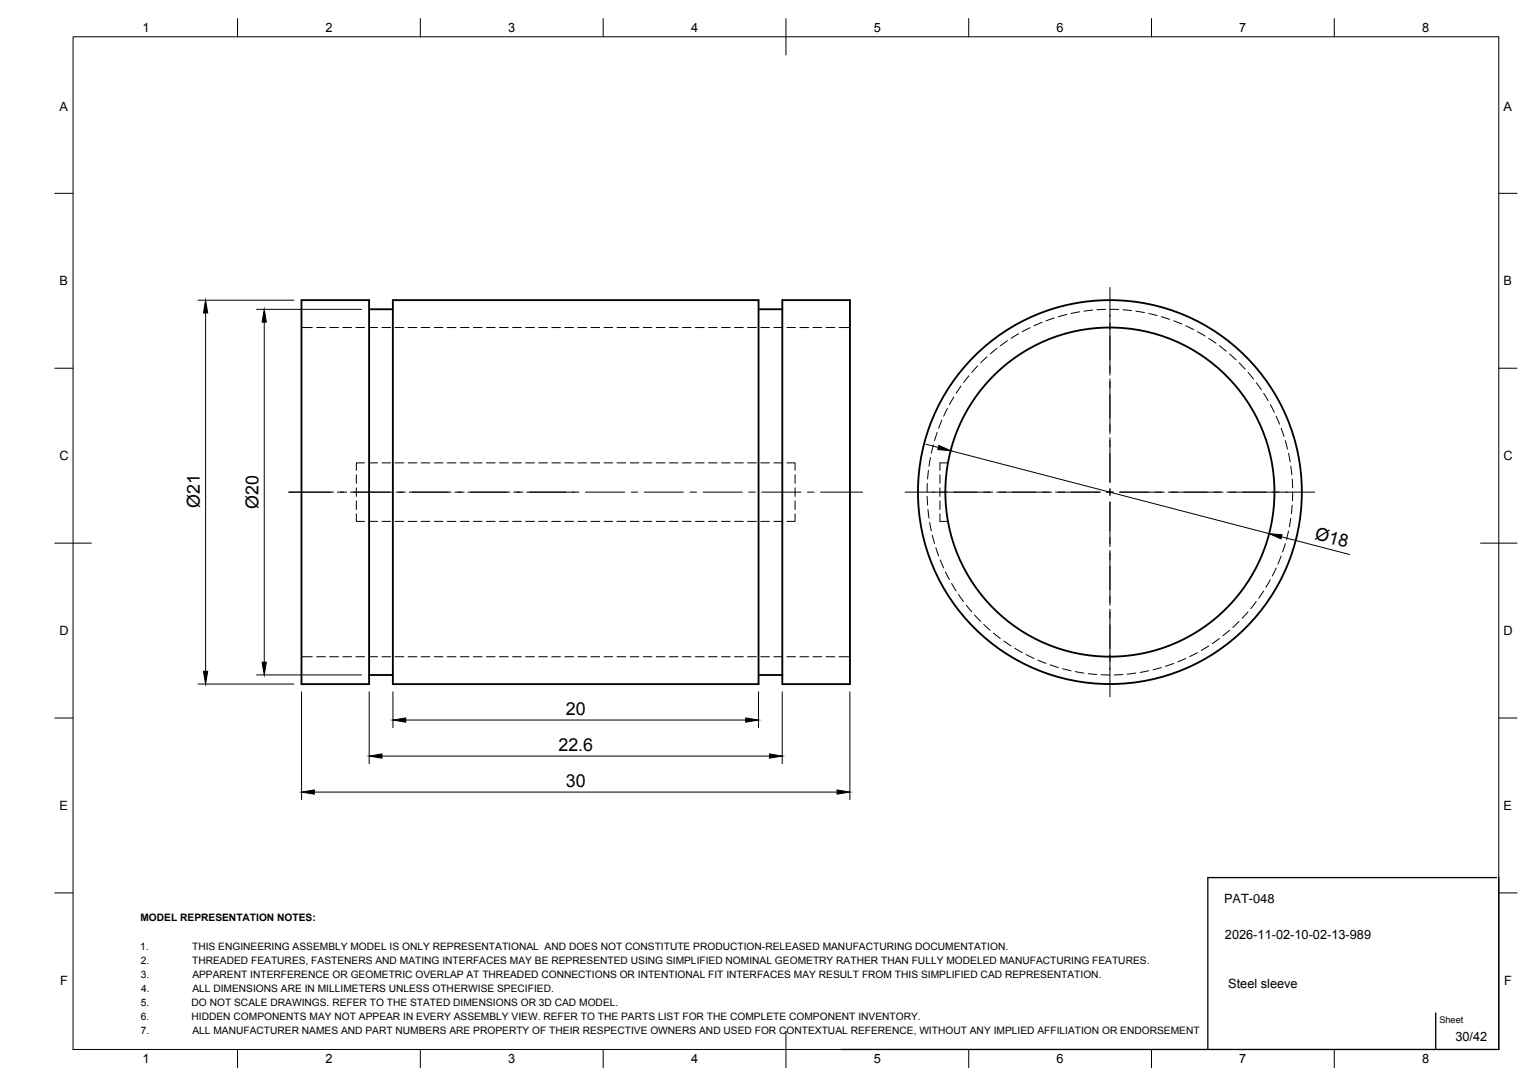
ISO-10303-21;
HEADER;
/* Generated by software containing ST-Developer
 * from STEP Tools, Inc. (www.steptools.com) 
 */

FILE_DESCRIPTION(
/* description */ ('Guided pneumatic stop gate'),
/* implementation_level */ '2;1');

FILE_NAME(
/* name */ 'Steel sleeve.step',
/* time_stamp */ '2026-10-27T21:43:45-07:00',
/* author */ (''),
/* organization */ (''),
/* preprocessor_version */ 'ST-DEVELOPER v20.2',
/* originating_system */ 'Autodesk Translation Framework v15.17.0.0',
/* authorisation */ '');

FILE_SCHEMA (('AUTOMOTIVE_DESIGN { 1 0 10303 214 3 1 1 }'));
ENDSEC;

DATA;
#10=MECHANICAL_DESIGN_GEOMETRIC_PRESENTATION_REPRESENTATION('',(#559),#14392);
#475=SHAPE_REPRESENTATION_RELATIONSHIP('SRR','None',#14611,#517);
#517=ADVANCED_BREP_SHAPE_REPRESENTATION('',(#600),#14373);
#559=STYLED_ITEM('',(#14905),#600);
#600=MANIFOLD_SOLID_BREP('Body1',#7900);
#777=FACE_BOUND('',#2059,.T.);
#778=FACE_BOUND('',#2062,.T.);
#779=FACE_BOUND('',#2065,.T.);
#780=FACE_BOUND('',#2068,.T.);
#781=FACE_BOUND('',#2071,.T.);
#782=FACE_BOUND('',#2074,.T.);
#783=FACE_BOUND('',#2076,.T.);
#1003=PLANE('',#8982);
#1004=PLANE('',#8984);
#1005=PLANE('',#8985);
#1006=PLANE('',#8987);
#1007=PLANE('',#8988);
#1008=PLANE('',#8989);
#1009=PLANE('',#8994);
#1010=PLANE('',#8998);
#1011=PLANE('',#9002);
#1012=PLANE('',#9006);
#1013=PLANE('',#9010);
#1416=FACE_OUTER_BOUND('',#2053,.T.);
#1417=FACE_OUTER_BOUND('',#2054,.T.);
#1418=FACE_OUTER_BOUND('',#2055,.T.);
#1419=FACE_OUTER_BOUND('',#2056,.T.);
#1420=FACE_OUTER_BOUND('',#2057,.T.);
#1421=FACE_OUTER_BOUND('',#2058,.T.);
#1422=FACE_OUTER_BOUND('',#2060,.T.);
#1423=FACE_OUTER_BOUND('',#2061,.T.);
#1424=FACE_OUTER_BOUND('',#2063,.T.);
#1425=FACE_OUTER_BOUND('',#2064,.T.);
#1426=FACE_OUTER_BOUND('',#2066,.T.);
#1427=FACE_OUTER_BOUND('',#2067,.T.);
#1428=FACE_OUTER_BOUND('',#2069,.T.);
#1429=FACE_OUTER_BOUND('',#2070,.T.);
#1430=FACE_OUTER_BOUND('',#2072,.T.);
#1431=FACE_OUTER_BOUND('',#2073,.T.);
#1432=FACE_OUTER_BOUND('',#2075,.T.);
#2053=EDGE_LOOP('',(#6546,#6547,#6548,#6549));
#2054=EDGE_LOOP('',(#6550,#6551,#6552,#6553));
#2055=EDGE_LOOP('',(#6554,#6555,#6556,#6557));
#2056=EDGE_LOOP('',(#6558,#6559,#6560,#6561));
#2057=EDGE_LOOP('',(#6562,#6563,#6564,#6565));
#2058=EDGE_LOOP('',(#6566));
#2059=EDGE_LOOP('',(#6567));
#2060=EDGE_LOOP('',(#6568,#6569,#6570,#6571));
#2061=EDGE_LOOP('',(#6572));
#2062=EDGE_LOOP('',(#6573));
#2063=EDGE_LOOP('',(#6574,#6575,#6576,#6577));
#2064=EDGE_LOOP('',(#6578));
#2065=EDGE_LOOP('',(#6579));
#2066=EDGE_LOOP('',(#6580,#6581,#6582,#6583));
#2067=EDGE_LOOP('',(#6584));
#2068=EDGE_LOOP('',(#6585));
#2069=EDGE_LOOP('',(#6586,#6587,#6588,#6589));
#2070=EDGE_LOOP('',(#6590));
#2071=EDGE_LOOP('',(#6591));
#2072=EDGE_LOOP('',(#6592,#6593,#6594,#6595));
#2073=EDGE_LOOP('',(#6596));
#2074=EDGE_LOOP('',(#6597));
#2075=EDGE_LOOP('',(#6598,#6599,#6600,#6601));
#2076=EDGE_LOOP('',(#6602,#6603,#6604,#6605));
#2612=LINE('',#13288,#3157);
#2613=LINE('',#13290,#3158);
#2614=LINE('',#13291,#3159);
#2615=LINE('',#13294,#3160);
#2616=LINE('',#13296,#3161);
#2617=LINE('',#13297,#3162);
#2618=LINE('',#13302,#3163);
#2619=LINE('',#13303,#3164);
#2620=LINE('',#13305,#3165);
#2621=LINE('',#13306,#3166);
#2622=LINE('',#13316,#3167);
#2623=LINE('',#13323,#3168);
#2624=LINE('',#13330,#3169);
#2625=LINE('',#13337,#3170);
#2626=LINE('',#13344,#3171);
#2627=LINE('',#13349,#3172);
#3157=VECTOR('',#10915,1.);
#3158=VECTOR('',#10916,1.);
#3159=VECTOR('',#10917,1.);
#3160=VECTOR('',#10920,1.);
#3161=VECTOR('',#10921,1.);
#3162=VECTOR('',#10922,1.);
#3163=VECTOR('',#10927,1.);
#3164=VECTOR('',#10928,1.);
#3165=VECTOR('',#10931,1.);
#3166=VECTOR('',#10932,1.);
#3167=VECTOR('',#10945,1.05);
#3168=VECTOR('',#10954,1.);
#3169=VECTOR('',#10963,1.05);
#3170=VECTOR('',#10972,1.);
#3171=VECTOR('',#10981,1.05);
#3172=VECTOR('',#10988,0.9);
#3623=CIRCLE('',#8983,0.9);
#3624=CIRCLE('',#8986,0.9);
#3625=CIRCLE('',#8990,1.05);
#3626=CIRCLE('',#8991,0.9);
#3627=CIRCLE('',#8993,1.05);
#3628=CIRCLE('',#8995,1.);
#3629=CIRCLE('',#8997,1.);
#3630=CIRCLE('',#8999,1.05);
#3631=CIRCLE('',#9001,1.05);
#3632=CIRCLE('',#9003,1.);
#3633=CIRCLE('',#9005,1.);
#3634=CIRCLE('',#9007,1.05);
#3635=CIRCLE('',#9009,1.05);
#3636=CIRCLE('',#9011,0.9);
#4132=VERTEX_POINT('',#13284);
#4133=VERTEX_POINT('',#13285);
#4134=VERTEX_POINT('',#13287);
#4135=VERTEX_POINT('',#13289);
#4136=VERTEX_POINT('',#13293);
#4137=VERTEX_POINT('',#13295);
#4138=VERTEX_POINT('',#13299);
#4139=VERTEX_POINT('',#13301);
#4140=VERTEX_POINT('',#13309);
#4141=VERTEX_POINT('',#13311);
#4142=VERTEX_POINT('',#13314);
#4143=VERTEX_POINT('',#13318);
#4144=VERTEX_POINT('',#13321);
#4145=VERTEX_POINT('',#13325);
#4146=VERTEX_POINT('',#13328);
#4147=VERTEX_POINT('',#13332);
#4148=VERTEX_POINT('',#13335);
#4149=VERTEX_POINT('',#13339);
#4150=VERTEX_POINT('',#13342);
#4151=VERTEX_POINT('',#13346);
#4971=EDGE_CURVE('',#4132,#4133,#3623,.T.);
#4972=EDGE_CURVE('',#4134,#4132,#2612,.T.);
#4973=EDGE_CURVE('',#4135,#4134,#2613,.T.);
#4974=EDGE_CURVE('',#4133,#4135,#2614,.T.);
#4975=EDGE_CURVE('',#4133,#4136,#2615,.T.);
#4976=EDGE_CURVE('',#4137,#4135,#2616,.T.);
#4977=EDGE_CURVE('',#4137,#4136,#2617,.T.);
#4978=EDGE_CURVE('',#4136,#4138,#3624,.T.);
#4979=EDGE_CURVE('',#4139,#4137,#2618,.T.);
#4980=EDGE_CURVE('',#4138,#4139,#2619,.T.);
#4981=EDGE_CURVE('',#4138,#4132,#2620,.T.);
#4982=EDGE_CURVE('',#4139,#4134,#2621,.T.);
#4983=EDGE_CURVE('',#4140,#4140,#3625,.T.);
#4984=EDGE_CURVE('',#4141,#4141,#3626,.T.);
#4985=EDGE_CURVE('',#4142,#4142,#3627,.T.);
#4986=EDGE_CURVE('',#4142,#4140,#2622,.T.);
#4987=EDGE_CURVE('',#4143,#4143,#3628,.T.);
#4988=EDGE_CURVE('',#4144,#4144,#3629,.T.);
#4989=EDGE_CURVE('',#4144,#4143,#2623,.T.);
#4990=EDGE_CURVE('',#4145,#4145,#3630,.T.);
#4991=EDGE_CURVE('',#4146,#4146,#3631,.T.);
#4992=EDGE_CURVE('',#4146,#4145,#2624,.T.);
#4993=EDGE_CURVE('',#4147,#4147,#3632,.T.);
#4994=EDGE_CURVE('',#4148,#4148,#3633,.T.);
#4995=EDGE_CURVE('',#4148,#4147,#2625,.T.);
#4996=EDGE_CURVE('',#4149,#4149,#3634,.T.);
#4997=EDGE_CURVE('',#4150,#4150,#3635,.T.);
#4998=EDGE_CURVE('',#4150,#4149,#2626,.T.);
#4999=EDGE_CURVE('',#4151,#4151,#3636,.T.);
#5000=EDGE_CURVE('',#4151,#4141,#2627,.T.);
#6546=ORIENTED_EDGE('',*,*,#4971,.F.);
#6547=ORIENTED_EDGE('',*,*,#4972,.F.);
#6548=ORIENTED_EDGE('',*,*,#4973,.F.);
#6549=ORIENTED_EDGE('',*,*,#4974,.F.);
#6550=ORIENTED_EDGE('',*,*,#4975,.F.);
#6551=ORIENTED_EDGE('',*,*,#4974,.T.);
#6552=ORIENTED_EDGE('',*,*,#4976,.F.);
#6553=ORIENTED_EDGE('',*,*,#4977,.T.);
#6554=ORIENTED_EDGE('',*,*,#4978,.F.);
#6555=ORIENTED_EDGE('',*,*,#4977,.F.);
#6556=ORIENTED_EDGE('',*,*,#4979,.F.);
#6557=ORIENTED_EDGE('',*,*,#4980,.F.);
#6558=ORIENTED_EDGE('',*,*,#4981,.F.);
#6559=ORIENTED_EDGE('',*,*,#4980,.T.);
#6560=ORIENTED_EDGE('',*,*,#4982,.T.);
#6561=ORIENTED_EDGE('',*,*,#4972,.T.);
#6562=ORIENTED_EDGE('',*,*,#4982,.F.);
#6563=ORIENTED_EDGE('',*,*,#4979,.T.);
#6564=ORIENTED_EDGE('',*,*,#4976,.T.);
#6565=ORIENTED_EDGE('',*,*,#4973,.T.);
#6566=ORIENTED_EDGE('',*,*,#4983,.F.);
#6567=ORIENTED_EDGE('',*,*,#4984,.T.);
#6568=ORIENTED_EDGE('',*,*,#4985,.F.);
#6569=ORIENTED_EDGE('',*,*,#4986,.T.);
#6570=ORIENTED_EDGE('',*,*,#4983,.T.);
#6571=ORIENTED_EDGE('',*,*,#4986,.F.);
#6572=ORIENTED_EDGE('',*,*,#4985,.T.);
#6573=ORIENTED_EDGE('',*,*,#4987,.F.);
#6574=ORIENTED_EDGE('',*,*,#4988,.F.);
#6575=ORIENTED_EDGE('',*,*,#4989,.T.);
#6576=ORIENTED_EDGE('',*,*,#4987,.T.);
#6577=ORIENTED_EDGE('',*,*,#4989,.F.);
#6578=ORIENTED_EDGE('',*,*,#4990,.F.);
#6579=ORIENTED_EDGE('',*,*,#4988,.T.);
#6580=ORIENTED_EDGE('',*,*,#4991,.F.);
#6581=ORIENTED_EDGE('',*,*,#4992,.T.);
#6582=ORIENTED_EDGE('',*,*,#4990,.T.);
#6583=ORIENTED_EDGE('',*,*,#4992,.F.);
#6584=ORIENTED_EDGE('',*,*,#4991,.T.);
#6585=ORIENTED_EDGE('',*,*,#4993,.F.);
#6586=ORIENTED_EDGE('',*,*,#4994,.F.);
#6587=ORIENTED_EDGE('',*,*,#4995,.T.);
#6588=ORIENTED_EDGE('',*,*,#4993,.T.);
#6589=ORIENTED_EDGE('',*,*,#4995,.F.);
#6590=ORIENTED_EDGE('',*,*,#4996,.F.);
#6591=ORIENTED_EDGE('',*,*,#4994,.T.);
#6592=ORIENTED_EDGE('',*,*,#4997,.F.);
#6593=ORIENTED_EDGE('',*,*,#4998,.T.);
#6594=ORIENTED_EDGE('',*,*,#4996,.T.);
#6595=ORIENTED_EDGE('',*,*,#4998,.F.);
#6596=ORIENTED_EDGE('',*,*,#4997,.T.);
#6597=ORIENTED_EDGE('',*,*,#4999,.F.);
#6598=ORIENTED_EDGE('',*,*,#4999,.T.);
#6599=ORIENTED_EDGE('',*,*,#5000,.T.);
#6600=ORIENTED_EDGE('',*,*,#4984,.F.);
#6601=ORIENTED_EDGE('',*,*,#5000,.F.);
#6602=ORIENTED_EDGE('',*,*,#4978,.T.);
#6603=ORIENTED_EDGE('',*,*,#4981,.T.);
#6604=ORIENTED_EDGE('',*,*,#4971,.T.);
#6605=ORIENTED_EDGE('',*,*,#4975,.T.);
#7357=CYLINDRICAL_SURFACE('',#8992,1.05);
#7358=CYLINDRICAL_SURFACE('',#8996,1.);
#7359=CYLINDRICAL_SURFACE('',#9000,1.05);
#7360=CYLINDRICAL_SURFACE('',#9004,1.);
#7361=CYLINDRICAL_SURFACE('',#9008,1.05);
#7362=CYLINDRICAL_SURFACE('',#9012,0.9);
#7698=ADVANCED_FACE('',(#1416),#1003,.F.);
#7699=ADVANCED_FACE('',(#1417),#1004,.F.);
#7700=ADVANCED_FACE('',(#1418),#1005,.F.);
#7701=ADVANCED_FACE('',(#1419),#1006,.F.);
#7702=ADVANCED_FACE('',(#1420),#1007,.F.);
#7703=ADVANCED_FACE('',(#1421,#777),#1008,.T.);
#7704=ADVANCED_FACE('',(#1422),#7357,.T.);
#7705=ADVANCED_FACE('',(#1423,#778),#1009,.T.);
#7706=ADVANCED_FACE('',(#1424),#7358,.T.);
#7707=ADVANCED_FACE('',(#1425,#779),#1010,.T.);
#7708=ADVANCED_FACE('',(#1426),#7359,.T.);
#7709=ADVANCED_FACE('',(#1427,#780),#1011,.T.);
#7710=ADVANCED_FACE('',(#1428),#7360,.T.);
#7711=ADVANCED_FACE('',(#1429,#781),#1012,.T.);
#7712=ADVANCED_FACE('',(#1430),#7361,.T.);
#7713=ADVANCED_FACE('',(#1431,#782),#1013,.T.);
#7714=ADVANCED_FACE('',(#1432,#783),#7362,.F.);
#7900=CLOSED_SHELL('',(#7698,#7699,#7700,#7701,#7702,#7703,#7704,#7705,
#7706,#7707,#7708,#7709,#7710,#7711,#7712,#7713,#7714));
#8981=AXIS2_PLACEMENT_3D('',#13282,#10909,#10910);
#8982=AXIS2_PLACEMENT_3D('',#13283,#10911,#10912);
#8983=AXIS2_PLACEMENT_3D('',#13286,#10913,#10914);
#8984=AXIS2_PLACEMENT_3D('',#13292,#10918,#10919);
#8985=AXIS2_PLACEMENT_3D('',#13298,#10923,#10924);
#8986=AXIS2_PLACEMENT_3D('',#13300,#10925,#10926);
#8987=AXIS2_PLACEMENT_3D('',#13304,#10929,#10930);
#8988=AXIS2_PLACEMENT_3D('',#13307,#10933,#10934);
#8989=AXIS2_PLACEMENT_3D('',#13308,#10935,#10936);
#8990=AXIS2_PLACEMENT_3D('',#13310,#10937,#10938);
#8991=AXIS2_PLACEMENT_3D('',#13312,#10939,#10940);
#8992=AXIS2_PLACEMENT_3D('',#13313,#10941,#10942);
#8993=AXIS2_PLACEMENT_3D('',#13315,#10943,#10944);
#8994=AXIS2_PLACEMENT_3D('',#13317,#10946,#10947);
#8995=AXIS2_PLACEMENT_3D('',#13319,#10948,#10949);
#8996=AXIS2_PLACEMENT_3D('',#13320,#10950,#10951);
#8997=AXIS2_PLACEMENT_3D('',#13322,#10952,#10953);
#8998=AXIS2_PLACEMENT_3D('',#13324,#10955,#10956);
#8999=AXIS2_PLACEMENT_3D('',#13326,#10957,#10958);
#9000=AXIS2_PLACEMENT_3D('',#13327,#10959,#10960);
#9001=AXIS2_PLACEMENT_3D('',#13329,#10961,#10962);
#9002=AXIS2_PLACEMENT_3D('',#13331,#10964,#10965);
#9003=AXIS2_PLACEMENT_3D('',#13333,#10966,#10967);
#9004=AXIS2_PLACEMENT_3D('',#13334,#10968,#10969);
#9005=AXIS2_PLACEMENT_3D('',#13336,#10970,#10971);
#9006=AXIS2_PLACEMENT_3D('',#13338,#10973,#10974);
#9007=AXIS2_PLACEMENT_3D('',#13340,#10975,#10976);
#9008=AXIS2_PLACEMENT_3D('',#13341,#10977,#10978);
#9009=AXIS2_PLACEMENT_3D('',#13343,#10979,#10980);
#9010=AXIS2_PLACEMENT_3D('',#13345,#10982,#10983);
#9011=AXIS2_PLACEMENT_3D('',#13347,#10984,#10985);
#9012=AXIS2_PLACEMENT_3D('',#13348,#10986,#10987);
#10909=DIRECTION('axis',(0.,0.,1.));
#10910=DIRECTION('refdir',(1.,0.,0.));
#10911=DIRECTION('center_axis',(0.,1.,0.));
#10912=DIRECTION('ref_axis',(0.,0.,1.));
#10913=DIRECTION('center_axis',(0.,-1.,0.));
#10914=DIRECTION('ref_axis',(1.,0.,0.));
#10915=DIRECTION('',(-1.,0.,0.));
#10916=DIRECTION('',(0.,0.,-1.));
#10917=DIRECTION('',(1.,0.,0.));
#10918=DIRECTION('center_axis',(0.,0.,1.));
#10919=DIRECTION('ref_axis',(1.,0.,0.));
#10920=DIRECTION('',(0.,-1.,0.));
#10921=DIRECTION('',(0.,1.,0.));
#10922=DIRECTION('',(-1.,0.,0.));
#10923=DIRECTION('center_axis',(0.,-1.,0.));
#10924=DIRECTION('ref_axis',(0.,0.,-1.));
#10925=DIRECTION('center_axis',(0.,1.,0.));
#10926=DIRECTION('ref_axis',(1.,0.,0.));
#10927=DIRECTION('',(0.,0.,1.));
#10928=DIRECTION('',(1.,0.,0.));
#10929=DIRECTION('center_axis',(0.,0.,-1.));
#10930=DIRECTION('ref_axis',(-1.,0.,0.));
#10931=DIRECTION('',(0.,1.,0.));
#10932=DIRECTION('',(0.,1.,0.));
#10933=DIRECTION('center_axis',(1.,0.,0.));
#10934=DIRECTION('ref_axis',(0.,0.,-1.));
#10935=DIRECTION('center_axis',(0.,1.,0.));
#10936=DIRECTION('ref_axis',(0.,0.,1.));
#10937=DIRECTION('center_axis',(0.,-1.,0.));
#10938=DIRECTION('ref_axis',(1.,0.,0.));
#10939=DIRECTION('center_axis',(0.,-1.,0.));
#10940=DIRECTION('ref_axis',(1.,0.,0.));
#10941=DIRECTION('center_axis',(0.,-1.,0.));
#10942=DIRECTION('ref_axis',(1.,0.,0.));
#10943=DIRECTION('center_axis',(0.,-1.,0.));
#10944=DIRECTION('ref_axis',(1.,0.,0.));
#10945=DIRECTION('',(0.,1.,0.));
#10946=DIRECTION('center_axis',(0.,-1.,0.));
#10947=DIRECTION('ref_axis',(0.,0.,-1.));
#10948=DIRECTION('center_axis',(0.,-1.,0.));
#10949=DIRECTION('ref_axis',(1.,0.,0.));
#10950=DIRECTION('center_axis',(0.,-1.,0.));
#10951=DIRECTION('ref_axis',(1.,0.,0.));
#10952=DIRECTION('center_axis',(0.,-1.,0.));
#10953=DIRECTION('ref_axis',(1.,0.,0.));
#10954=DIRECTION('',(0.,1.,0.));
#10955=DIRECTION('center_axis',(0.,1.,0.));
#10956=DIRECTION('ref_axis',(0.,0.,1.));
#10957=DIRECTION('center_axis',(0.,-1.,0.));
#10958=DIRECTION('ref_axis',(1.,0.,0.));
#10959=DIRECTION('center_axis',(0.,-1.,0.));
#10960=DIRECTION('ref_axis',(1.,0.,0.));
#10961=DIRECTION('center_axis',(0.,-1.,0.));
#10962=DIRECTION('ref_axis',(1.,0.,0.));
#10963=DIRECTION('',(0.,1.,0.));
#10964=DIRECTION('center_axis',(0.,-1.,0.));
#10965=DIRECTION('ref_axis',(0.,0.,-1.));
#10966=DIRECTION('center_axis',(0.,-1.,0.));
#10967=DIRECTION('ref_axis',(1.,0.,0.));
#10968=DIRECTION('center_axis',(0.,-1.,0.));
#10969=DIRECTION('ref_axis',(1.,0.,0.));
#10970=DIRECTION('center_axis',(0.,-1.,0.));
#10971=DIRECTION('ref_axis',(1.,0.,0.));
#10972=DIRECTION('',(0.,1.,0.));
#10973=DIRECTION('center_axis',(0.,1.,0.));
#10974=DIRECTION('ref_axis',(0.,0.,1.));
#10975=DIRECTION('center_axis',(0.,-1.,0.));
#10976=DIRECTION('ref_axis',(1.,0.,0.));
#10977=DIRECTION('center_axis',(0.,-1.,0.));
#10978=DIRECTION('ref_axis',(1.,0.,0.));
#10979=DIRECTION('center_axis',(0.,-1.,0.));
#10980=DIRECTION('ref_axis',(1.,0.,0.));
#10981=DIRECTION('',(0.,1.,0.));
#10982=DIRECTION('center_axis',(0.,-1.,0.));
#10983=DIRECTION('ref_axis',(0.,0.,-1.));
#10984=DIRECTION('center_axis',(0.,-1.,0.));
#10985=DIRECTION('ref_axis',(1.,0.,0.));
#10986=DIRECTION('center_axis',(0.,-1.,0.));
#10987=DIRECTION('ref_axis',(1.,0.,0.));
#10988=DIRECTION('',(0.,1.,0.));
#13282=CARTESIAN_POINT('',(0.,0.,0.));
#13283=CARTESIAN_POINT('Origin',(0.75,1.2,0.));
#13284=CARTESIAN_POINT('',(0.885663593019381,1.2,-0.16));
#13285=CARTESIAN_POINT('',(0.885663593019381,1.2,0.16));
#13286=CARTESIAN_POINT('Origin',(0.,1.2,0.));
#13287=CARTESIAN_POINT('',(0.93,1.2,-0.16));
#13288=CARTESIAN_POINT('',(0.93,1.2,-0.16));
#13289=CARTESIAN_POINT('',(0.93,1.2,0.16));
#13290=CARTESIAN_POINT('',(0.93,1.2,0.16));
#13291=CARTESIAN_POINT('',(0.57,1.2,0.16));
#13292=CARTESIAN_POINT('Origin',(0.57,0.,0.16));
#13293=CARTESIAN_POINT('',(0.885663593019381,-1.2,0.16));
#13294=CARTESIAN_POINT('',(0.885663593019381,0.,0.16));
#13295=CARTESIAN_POINT('',(0.93,-1.2,0.16));
#13296=CARTESIAN_POINT('',(0.93,0.,0.16));
#13297=CARTESIAN_POINT('',(0.57,-1.2,0.16));
#13298=CARTESIAN_POINT('Origin',(0.75,-1.2,0.));
#13299=CARTESIAN_POINT('',(0.885663593019381,-1.2,-0.16));
#13300=CARTESIAN_POINT('Origin',(0.,-1.2,0.));
#13301=CARTESIAN_POINT('',(0.93,-1.2,-0.16));
#13302=CARTESIAN_POINT('',(0.93,-1.2,0.16));
#13303=CARTESIAN_POINT('',(0.93,-1.2,-0.16));
#13304=CARTESIAN_POINT('Origin',(0.93,0.,-0.16));
#13305=CARTESIAN_POINT('',(0.885663593019381,0.,-0.16));
#13306=CARTESIAN_POINT('',(0.93,0.,-0.16));
#13307=CARTESIAN_POINT('Origin',(0.93,0.,0.16));
#13308=CARTESIAN_POINT('Origin',(1.05,1.5,0.));
#13309=CARTESIAN_POINT('',(-1.05,1.5,-1.28587913910472E-16));
#13310=CARTESIAN_POINT('Origin',(0.,1.5,0.));
#13311=CARTESIAN_POINT('',(-0.9,1.5,-1.10218211923262E-16));
#13312=CARTESIAN_POINT('Origin',(0.,1.5,0.));
#13313=CARTESIAN_POINT('Origin',(0.,1.315,0.));
#13314=CARTESIAN_POINT('',(-1.05,1.13,-1.28587913910472E-16));
#13315=CARTESIAN_POINT('Origin',(0.,1.13,0.));
#13316=CARTESIAN_POINT('',(-1.05,1.315,-1.28587913910472E-16));
#13317=CARTESIAN_POINT('Origin',(1.,1.13,0.));
#13318=CARTESIAN_POINT('',(-1.,1.13,-1.22464679914735E-16));
#13319=CARTESIAN_POINT('Origin',(0.,1.13,0.));
#13320=CARTESIAN_POINT('Origin',(0.,1.065,0.));
#13321=CARTESIAN_POINT('',(-1.,1.,-1.22464679914735E-16));
#13322=CARTESIAN_POINT('Origin',(0.,1.,0.));
#13323=CARTESIAN_POINT('',(-1.,1.065,-1.22464679914735E-16));
#13324=CARTESIAN_POINT('Origin',(1.05,1.,0.));
#13325=CARTESIAN_POINT('',(-1.05,1.,-1.28587913910472E-16));
#13326=CARTESIAN_POINT('Origin',(0.,1.,0.));
#13327=CARTESIAN_POINT('Origin',(0.,0.,0.));
#13328=CARTESIAN_POINT('',(-1.05,-1.,-1.28587913910472E-16));
#13329=CARTESIAN_POINT('Origin',(0.,-1.,0.));
#13330=CARTESIAN_POINT('',(-1.05,0.,-1.28587913910472E-16));
#13331=CARTESIAN_POINT('Origin',(1.,-1.,0.));
#13332=CARTESIAN_POINT('',(-1.,-1.,-1.22464679914735E-16));
#13333=CARTESIAN_POINT('Origin',(0.,-1.,0.));
#13334=CARTESIAN_POINT('Origin',(0.,-1.065,0.));
#13335=CARTESIAN_POINT('',(-1.,-1.13,-1.22464679914735E-16));
#13336=CARTESIAN_POINT('Origin',(0.,-1.13,0.));
#13337=CARTESIAN_POINT('',(-1.,-1.065,-1.22464679914735E-16));
#13338=CARTESIAN_POINT('Origin',(1.05,-1.13,0.));
#13339=CARTESIAN_POINT('',(-1.05,-1.13,-1.28587913910472E-16));
#13340=CARTESIAN_POINT('Origin',(0.,-1.13,0.));
#13341=CARTESIAN_POINT('Origin',(0.,-1.315,0.));
#13342=CARTESIAN_POINT('',(-1.05,-1.5,-1.28587913910472E-16));
#13343=CARTESIAN_POINT('Origin',(0.,-1.5,0.));
#13344=CARTESIAN_POINT('',(-1.05,-1.315,-1.28587913910472E-16));
#13345=CARTESIAN_POINT('Origin',(0.9,-1.5,0.));
#13346=CARTESIAN_POINT('',(-0.9,-1.5,-1.10218211923262E-16));
#13347=CARTESIAN_POINT('Origin',(0.,-1.5,0.));
#13348=CARTESIAN_POINT('Origin',(0.,0.,0.));
#13349=CARTESIAN_POINT('',(-0.9,0.,-1.10218211923262E-16));
#14325=UNCERTAINTY_MEASURE_WITH_UNIT(LENGTH_MEASURE(0.001),#14393,
'DISTANCE_ACCURACY_VALUE',
'Maximum model space distance between geometric entities at asserted c
onnectivities');
#14344=UNCERTAINTY_MEASURE_WITH_UNIT(LENGTH_MEASURE(0.001),#14393,
'DISTANCE_ACCURACY_VALUE',
'Maximum model space distance between geometric entities at asserted c
onnectivities');
#14373=(
GEOMETRIC_REPRESENTATION_CONTEXT(3)
GLOBAL_UNCERTAINTY_ASSIGNED_CONTEXT((#14325))
GLOBAL_UNIT_ASSIGNED_CONTEXT((#14393,#14395,#14396))
REPRESENTATION_CONTEXT('','3D')
);
#14392=(
GEOMETRIC_REPRESENTATION_CONTEXT(3)
GLOBAL_UNCERTAINTY_ASSIGNED_CONTEXT((#14344))
GLOBAL_UNIT_ASSIGNED_CONTEXT((#14393,#14395,#14396))
REPRESENTATION_CONTEXT('','3D')
);
#14393=(
LENGTH_UNIT()
NAMED_UNIT(*)
SI_UNIT(.CENTI.,.METRE.)
);
#14395=(
NAMED_UNIT(*)
PLANE_ANGLE_UNIT()
SI_UNIT($,.RADIAN.)
);
#14396=(
NAMED_UNIT(*)
SI_UNIT($,.STERADIAN.)
SOLID_ANGLE_UNIT()
);
#14425=SHAPE_DEFINITION_REPRESENTATION(#14474,#14611);
#14474=PRODUCT_DEFINITION_SHAPE('',$,#14659);
#14611=SHAPE_REPRESENTATION('',(#8981),#14373);
#14630=PRODUCT_DEFINITION_CONTEXT('part definition',#14773,'design');
#14659=PRODUCT_DEFINITION('Steel sleeve','Steel sleeve',#14706,#14630);
#14706=PRODUCT_DEFINITION_FORMATION('',$,#14803);
#14773=APPLICATION_CONTEXT(
'Core Data for Automotive Mechanical Design Process');
#14774=PRODUCT_CONTEXT('part definition',#14773,'mechanical');
#14803=PRODUCT('Steel sleeve','Steel sleeve','Steel sleeve',(#14774));
#14899=COLOUR_RGB('Off White',0.89,0.88,0.83);
#14900=FILL_AREA_STYLE_COLOUR('',#14899);
#14901=FILL_AREA_STYLE('',(#14900));
#14902=SURFACE_STYLE_FILL_AREA(#14901);
#14903=SURFACE_SIDE_STYLE('',(#14902));
#14904=SURFACE_STYLE_USAGE(.BOTH.,#14903);
#14905=PRESENTATION_STYLE_ASSIGNMENT((#14904));
ENDSEC;
END-ISO-10303-21;
